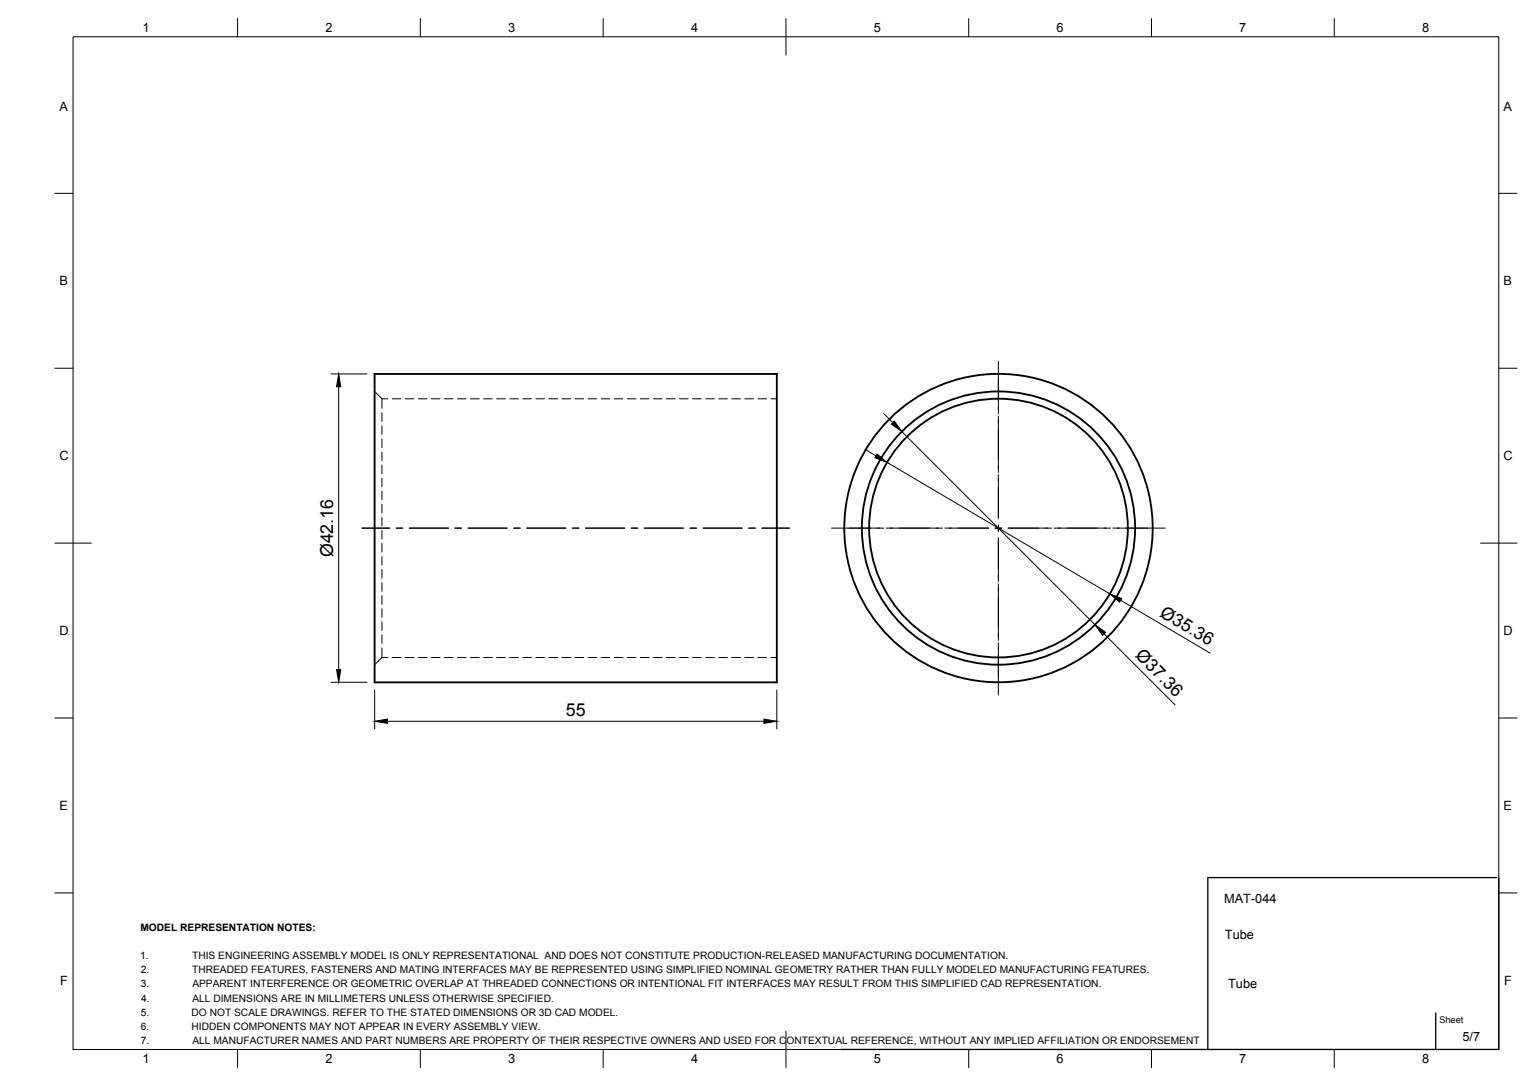
ISO-10303-21;
HEADER;
/* Generated by software containing ST-Developer
 * from STEP Tools, Inc. (www.steptools.com) 
 */

FILE_DESCRIPTION(
/* description */ ('STEP AP214'),
/* implementation_level */ '2;1');

FILE_NAME(
/* name */ 'Tube.step',
/* time_stamp */ '2026-11-14T22:20:24-08:00',
/* author */ (''),
/* organization */ (''),
/* preprocessor_version */ 'ST-DEVELOPER v20.2',
/* originating_system */ 'Autodesk Translation Framework v15.17.0.0',
/* authorisation */ '');

FILE_SCHEMA (('AUTOMOTIVE_DESIGN { 1 0 10303 214 3 1 1 }'));
ENDSEC;

DATA;
#10=MECHANICAL_DESIGN_GEOMETRIC_PRESENTATION_REPRESENTATION('',(#86),#2794);
#71=CONICAL_SURFACE('',#1830,18.6799999999998,0.785398163397447);
#76=SHAPE_REPRESENTATION_RELATIONSHIP('SRR','None',#2831,#81);
#81=ADVANCED_BREP_SHAPE_REPRESENTATION('',(#91),#2793);
#86=STYLED_ITEM('',(#2863),#91);
#91=MANIFOLD_SOLID_BREP('Body1',#1645);
#114=FACE_BOUND('',#389,.T.);
#115=FACE_BOUND('',#391,.T.);
#184=PLANE('',#1838);
#185=PLANE('',#1839);
#272=FACE_OUTER_BOUND('',#385,.T.);
#273=FACE_OUTER_BOUND('',#386,.T.);
#274=FACE_OUTER_BOUND('',#387,.T.);
#275=FACE_OUTER_BOUND('',#388,.T.);
#276=FACE_OUTER_BOUND('',#390,.T.);
#385=EDGE_LOOP('',(#1514,#1515,#1516,#1517));
#386=EDGE_LOOP('',(#1518,#1519,#1520,#1521));
#387=EDGE_LOOP('',(#1522,#1523,#1524,#1525));
#388=EDGE_LOOP('',(#1526));
#389=EDGE_LOOP('',(#1527));
#390=EDGE_LOOP('',(#1528));
#391=EDGE_LOOP('',(#1529));
#558=LINE('',#2752,#727);
#559=LINE('',#2757,#728);
#560=LINE('',#2762,#729);
#727=VECTOR('',#2281,18.6799999999998);
#728=VECTOR('',#2288,17.6799999999998);
#729=VECTOR('',#2293,21.0799999999997);
#766=CIRCLE('',#1831,17.6799999999998);
#767=CIRCLE('',#1832,18.6799999999998);
#768=CIRCLE('',#1834,17.6799999999998);
#769=CIRCLE('',#1836,21.0799999999997);
#770=CIRCLE('',#1837,21.0799999999997);
#895=VERTEX_POINT('',#2749);
#896=VERTEX_POINT('',#2751);
#897=VERTEX_POINT('',#2755);
#898=VERTEX_POINT('',#2759);
#899=VERTEX_POINT('',#2761);
#1102=EDGE_CURVE('',#895,#895,#766,.T.);
#1103=EDGE_CURVE('',#895,#896,#558,.T.);
#1104=EDGE_CURVE('',#896,#896,#767,.T.);
#1105=EDGE_CURVE('',#897,#897,#768,.T.);
#1106=EDGE_CURVE('',#897,#895,#559,.T.);
#1107=EDGE_CURVE('',#898,#898,#769,.T.);
#1108=EDGE_CURVE('',#898,#899,#560,.T.);
#1109=EDGE_CURVE('',#899,#899,#770,.T.);
#1514=ORIENTED_EDGE('',*,*,#1102,.F.);
#1515=ORIENTED_EDGE('',*,*,#1103,.T.);
#1516=ORIENTED_EDGE('',*,*,#1104,.F.);
#1517=ORIENTED_EDGE('',*,*,#1103,.F.);
#1518=ORIENTED_EDGE('',*,*,#1105,.T.);
#1519=ORIENTED_EDGE('',*,*,#1106,.T.);
#1520=ORIENTED_EDGE('',*,*,#1102,.T.);
#1521=ORIENTED_EDGE('',*,*,#1106,.F.);
#1522=ORIENTED_EDGE('',*,*,#1107,.T.);
#1523=ORIENTED_EDGE('',*,*,#1108,.T.);
#1524=ORIENTED_EDGE('',*,*,#1109,.F.);
#1525=ORIENTED_EDGE('',*,*,#1108,.F.);
#1526=ORIENTED_EDGE('',*,*,#1109,.T.);
#1527=ORIENTED_EDGE('',*,*,#1105,.F.);
#1528=ORIENTED_EDGE('',*,*,#1107,.F.);
#1529=ORIENTED_EDGE('',*,*,#1104,.T.);
#1548=CYLINDRICAL_SURFACE('',#1833,17.6799999999998);
#1549=CYLINDRICAL_SURFACE('',#1835,21.0799999999997);
#1636=ADVANCED_FACE('',(#272),#71,.F.);
#1637=ADVANCED_FACE('',(#273),#1548,.F.);
#1638=ADVANCED_FACE('',(#274),#1549,.T.);
#1639=ADVANCED_FACE('',(#275,#114),#184,.T.);
#1640=ADVANCED_FACE('',(#276,#115),#185,.F.);
#1645=CLOSED_SHELL('',(#1636,#1637,#1638,#1639,#1640));
#1829=AXIS2_PLACEMENT_3D('',#2747,#2275,#2276);
#1830=AXIS2_PLACEMENT_3D('',#2748,#2277,#2278);
#1831=AXIS2_PLACEMENT_3D('',#2750,#2279,#2280);
#1832=AXIS2_PLACEMENT_3D('',#2753,#2282,#2283);
#1833=AXIS2_PLACEMENT_3D('',#2754,#2284,#2285);
#1834=AXIS2_PLACEMENT_3D('',#2756,#2286,#2287);
#1835=AXIS2_PLACEMENT_3D('',#2758,#2289,#2290);
#1836=AXIS2_PLACEMENT_3D('',#2760,#2291,#2292);
#1837=AXIS2_PLACEMENT_3D('',#2763,#2294,#2295);
#1838=AXIS2_PLACEMENT_3D('',#2764,#2296,#2297);
#1839=AXIS2_PLACEMENT_3D('',#2765,#2298,#2299);
#2275=DIRECTION('axis',(0.,0.,1.));
#2276=DIRECTION('refdir',(1.,0.,0.));
#2277=DIRECTION('center_axis',(6.34239344602916E-18,1.46822901856177E-15,
-1.));
#2278=DIRECTION('ref_axis',(-1.,-3.13984949151806E-15,-6.34239344603377E-18));
#2279=DIRECTION('center_axis',(6.34239344602916E-18,1.46822901856177E-15,
-1.));
#2280=DIRECTION('ref_axis',(1.,3.13984949151806E-15,6.34239344603377E-18));
#2281=DIRECTION('',(0.707106781186546,3.1718079570939E-15,-0.707106781186549));
#2282=DIRECTION('center_axis',(-6.34239344602916E-18,-1.46822901856177E-15,
1.));
#2283=DIRECTION('ref_axis',(1.,3.13984949151806E-15,6.34239344603377E-18));
#2284=DIRECTION('center_axis',(6.34239344602916E-18,1.46822901856177E-15,
-1.));
#2285=DIRECTION('ref_axis',(-1.,-3.13984949151806E-15,-6.34239344603377E-18));
#2286=DIRECTION('center_axis',(-6.34239344602916E-18,-1.46822901856177E-15,
1.));
#2287=DIRECTION('ref_axis',(1.,3.13984949151806E-15,6.34239344603377E-18));
#2288=DIRECTION('',(6.34239344602916E-18,1.46822901856177E-15,-1.));
#2289=DIRECTION('center_axis',(6.34239344602916E-18,1.46822901856177E-15,
-1.));
#2290=DIRECTION('ref_axis',(-1.,-3.13984949151806E-15,-6.34239344603377E-18));
#2291=DIRECTION('center_axis',(-6.34239344602916E-18,-1.46822901856177E-15,
1.));
#2292=DIRECTION('ref_axis',(1.,3.13984949151806E-15,6.34239344603377E-18));
#2293=DIRECTION('',(-6.34239344602916E-18,-1.46822901856177E-15,1.));
#2294=DIRECTION('center_axis',(-6.34239344602916E-18,-1.46822901856177E-15,
1.));
#2295=DIRECTION('ref_axis',(1.,3.13984949151806E-15,6.34239344603377E-18));
#2296=DIRECTION('center_axis',(6.34239344603457E-18,-1.46822901856177E-15,
1.));
#2297=DIRECTION('ref_axis',(1.,3.13984949151806E-15,-6.34239344602996E-18));
#2298=DIRECTION('center_axis',(6.34239344603457E-18,-1.46822901856177E-15,
1.));
#2299=DIRECTION('ref_axis',(1.,3.13984949151806E-15,-6.34239344602996E-18));
#2747=CARTESIAN_POINT('',(0.,0.,0.));
#2748=CARTESIAN_POINT('Origin',(0.,0.,0.));
#2749=CARTESIAN_POINT('',(17.6799999999998,5.18791344505844E-14,0.999999999999992));
#2750=CARTESIAN_POINT('Origin',(0.,0.,0.999999999999994));
#2751=CARTESIAN_POINT('',(18.6799999999998,5.63647482807494E-14,-6.00207461602546E-16));
#2752=CARTESIAN_POINT('',(18.6799999999998,5.63647482807494E-14,1.18475909571906E-16));
#2753=CARTESIAN_POINT('Origin',(0.,0.,0.));
#2754=CARTESIAN_POINT('Origin',(0.,0.,54.9999999999998));
#2755=CARTESIAN_POINT('',(17.6799999999998,5.33473634691461E-14,54.9999999999998));
#2756=CARTESIAN_POINT('Origin',(0.,0.,54.9999999999998));
#2757=CARTESIAN_POINT('',(17.6799999999998,5.33473634691461E-14,54.9999999999998));
#2758=CARTESIAN_POINT('Origin',(0.,0.,54.9999999999998));
#2759=CARTESIAN_POINT('',(21.0799999999997,1.44359067849494E-13,0.));
#2760=CARTESIAN_POINT('Origin',(0.,0.,0.));
#2761=CARTESIAN_POINT('',(21.0799999999997,6.36064718285973E-14,54.9999999999998));
#2762=CARTESIAN_POINT('',(21.0799999999997,6.36064718285973E-14,54.9999999999998));
#2763=CARTESIAN_POINT('Origin',(0.,0.,54.9999999999998));
#2764=CARTESIAN_POINT('Origin',(0.,0.,54.9999999999998));
#2765=CARTESIAN_POINT('Origin',(0.,0.,0.));
#2786=UNCERTAINTY_MEASURE_WITH_UNIT(LENGTH_MEASURE(0.01),#2795,
'DISTANCE_ACCURACY_VALUE',
'Maximum model space distance between geometric entities at asserted c
onnectivities');
#2787=UNCERTAINTY_MEASURE_WITH_UNIT(LENGTH_MEASURE(0.01),#2795,
'DISTANCE_ACCURACY_VALUE',
'Maximum model space distance between geometric entities at asserted c
onnectivities');
#2793=(
GEOMETRIC_REPRESENTATION_CONTEXT(3)
GLOBAL_UNCERTAINTY_ASSIGNED_CONTEXT((#2786))
GLOBAL_UNIT_ASSIGNED_CONTEXT((#2795,#2797,#2798))
REPRESENTATION_CONTEXT('','3D')
);
#2794=(
GEOMETRIC_REPRESENTATION_CONTEXT(3)
GLOBAL_UNCERTAINTY_ASSIGNED_CONTEXT((#2787))
GLOBAL_UNIT_ASSIGNED_CONTEXT((#2795,#2797,#2798))
REPRESENTATION_CONTEXT('','3D')
);
#2795=(
LENGTH_UNIT()
NAMED_UNIT(*)
SI_UNIT(.MILLI.,.METRE.)
);
#2797=(
NAMED_UNIT(*)
PLANE_ANGLE_UNIT()
SI_UNIT($,.RADIAN.)
);
#2798=(
NAMED_UNIT(*)
SI_UNIT($,.STERADIAN.)
SOLID_ANGLE_UNIT()
);
#2804=SHAPE_DEFINITION_REPRESENTATION(#2810,#2831);
#2810=PRODUCT_DEFINITION_SHAPE('',$,#2838);
#2831=SHAPE_REPRESENTATION('',(#1829),#2793);
#2832=PRODUCT_DEFINITION_CONTEXT('part definition',#2852,'design');
#2838=PRODUCT_DEFINITION('Tube','Tube',#2844,#2832);
#2844=PRODUCT_DEFINITION_FORMATION('',$,#2859);
#2852=APPLICATION_CONTEXT(
'Core Data for Automotive Mechanical Design Process');
#2853=PRODUCT_CONTEXT('part definition',#2852,'mechanical');
#2859=PRODUCT('Tube','Tube',$,(#2853));
#2863=PRESENTATION_STYLE_ASSIGNMENT((#2867));
#2867=SURFACE_STYLE_USAGE(.BOTH.,#2871);
#2871=SURFACE_SIDE_STYLE('',(#2875));
#2875=SURFACE_STYLE_FILL_AREA(#2879);
#2879=FILL_AREA_STYLE('Opaque(227,224,212)',(#2883));
#2883=FILL_AREA_STYLE_COLOUR('Opaque(227,224,212)',#2887);
#2887=COLOUR_RGB('Opaque(227,224,212)',0.890196078431372,0.87843137254902,
0.831372549019608);
ENDSEC;
END-ISO-10303-21;
